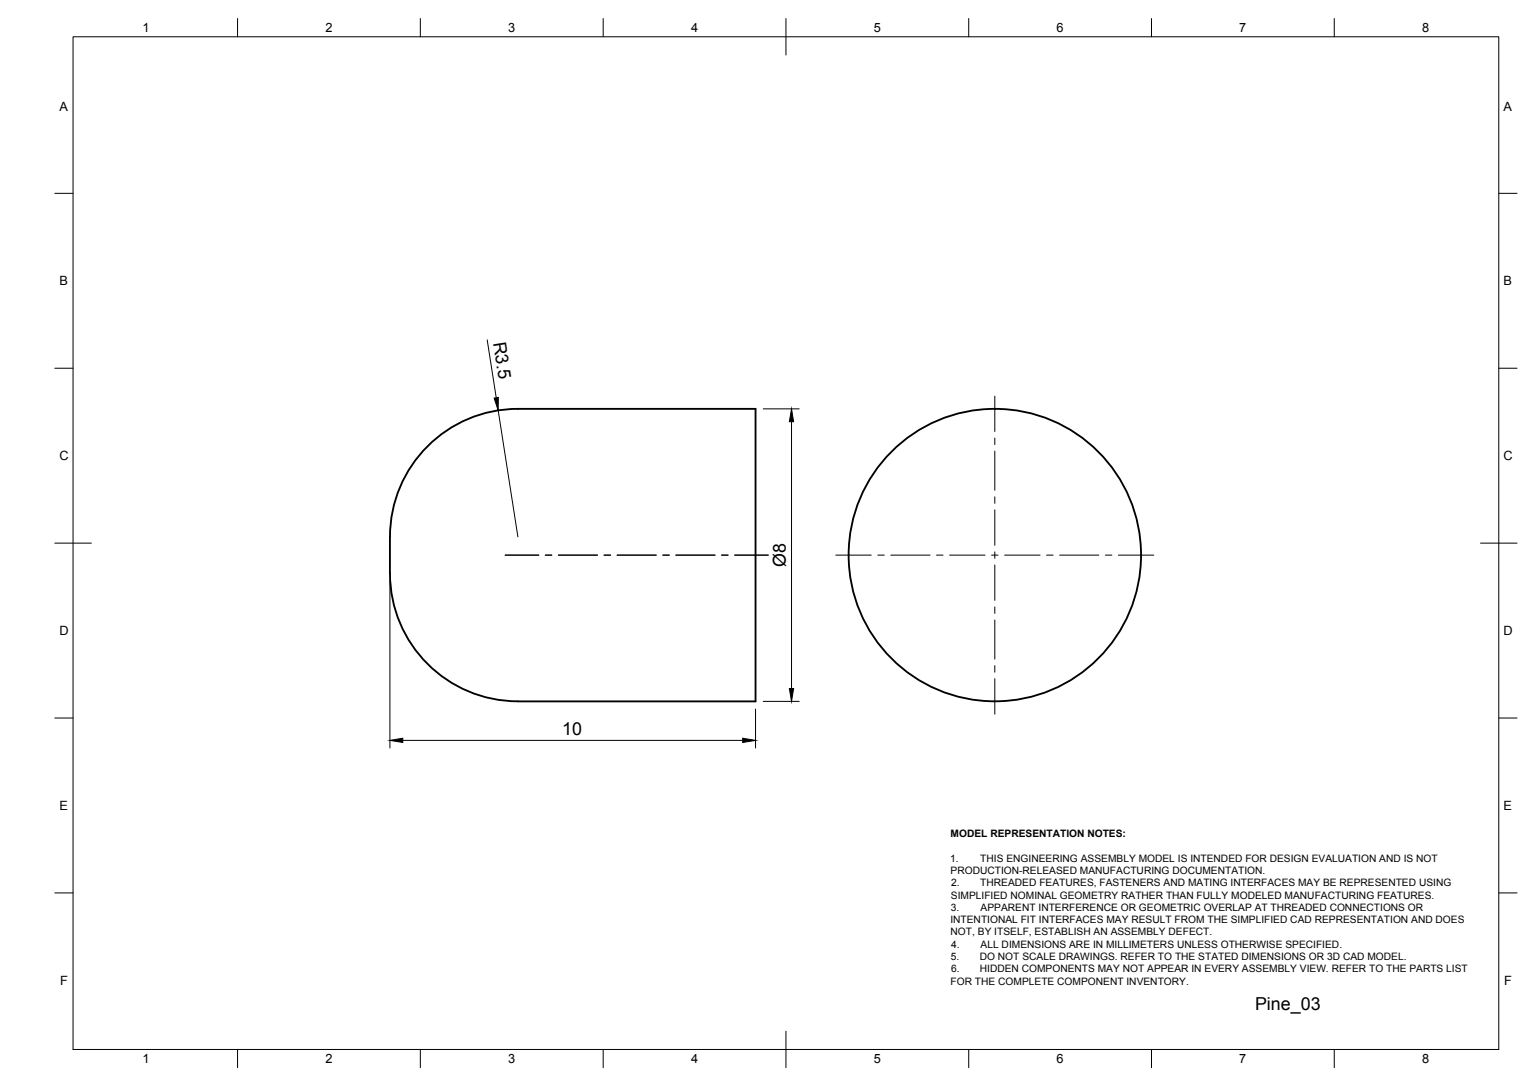
ISO-10303-21;
HEADER;
/* Generated by software containing ST-Developer
 * from STEP Tools, Inc. (www.steptools.com) 
 */

FILE_DESCRIPTION(
/* description */ (''),
/* implementation_level */ '2;1');

FILE_NAME(
/* name */ 'Pine_03.step',
/* time_stamp */ '2026-10-06T13:31:15-07:00',
/* author */ (''),
/* organization */ (''),
/* preprocessor_version */ 'ST-DEVELOPER v20.2',
/* originating_system */ 'Autodesk Translation Framework v15.15.0.0',
/* authorisation */ '');

FILE_SCHEMA (('AUTOMOTIVE_DESIGN { 1 0 10303 214 3 1 1 }'));
ENDSEC;

DATA;
#10=MECHANICAL_DESIGN_GEOMETRIC_PRESENTATION_REPRESENTATION('',(#84),#3154);
#49=(
BOUNDED_SURFACE()
B_SPLINE_SURFACE(2,2,((#2224,#2225,#2226,#2227,#2228,#2229,#2230,#2231,
#2232),(#2233,#2234,#2235,#2236,#2237,#2238,#2239,#2240,#2241),(#2242,#2243,
#2244,#2245,#2246,#2247,#2248,#2249,#2250)),.UNSPECIFIED.,.F.,.T.,.F.)
B_SPLINE_SURFACE_WITH_KNOTS((3,3),(3,2,2,2,3),(-6.11109985317371E-14,1.57079632679497),
(-3.14159265358979,-1.5707963267949,0.,1.5707963267949,3.14159265358979),
 .UNSPECIFIED.)
GEOMETRIC_REPRESENTATION_ITEM()
RATIONAL_B_SPLINE_SURFACE(((1.,0.707106781186548,1.,0.707106781186548,1.,
0.707106781186548,1.,0.707106781186548,1.),(0.707106781186505,0.49999999999997,
0.707106781186505,0.49999999999997,0.707106781186505,0.49999999999997,0.707106781186505,
0.49999999999997,0.707106781186505),(1.,0.707106781186548,1.,0.707106781186548,
1.,0.707106781186548,1.,0.707106781186548,1.)))
REPRESENTATION_ITEM('')
SURFACE()
);
#66=SHAPE_REPRESENTATION_RELATIONSHIP('SRR','None',#3194,#75);
#75=ADVANCED_BREP_SHAPE_REPRESENTATION('',(#93),#3150);
#84=STYLED_ITEM('',(#3243),#93);
#93=MANIFOLD_SOLID_BREP('Body1',#1086);
#114=PLANE('',#1246);
#115=PLANE('',#1247);
#157=CIRCLE('',#1240,3.99999999999999);
#158=CIRCLE('',#1241,3.49999999999999);
#159=CIRCLE('',#1242,0.49999999999999);
#160=CIRCLE('',#1243,3.99999999999999);
#161=CIRCLE('',#1245,3.99999999999999);
#202=FACE_OUTER_BOUND('',#266,.T.);
#203=FACE_OUTER_BOUND('',#267,.T.);
#204=FACE_OUTER_BOUND('',#268,.T.);
#205=FACE_OUTER_BOUND('',#269,.T.);
#266=EDGE_LOOP('',(#856,#857,#858,#859,#860));
#267=EDGE_LOOP('',(#861,#862,#863,#864,#865));
#268=EDGE_LOOP('',(#866));
#269=EDGE_LOOP('',(#867));
#332=LINE('',#2260,#398);
#398=VECTOR('',#1428,3.99999999999999);
#524=VERTEX_POINT('',#2251);
#525=VERTEX_POINT('',#2252);
#526=VERTEX_POINT('',#2254);
#527=VERTEX_POINT('',#2259);
#644=EDGE_CURVE('',#524,#525,#157,.T.);
#645=EDGE_CURVE('',#525,#526,#158,.T.);
#646=EDGE_CURVE('',#526,#526,#159,.T.);
#647=EDGE_CURVE('',#525,#524,#160,.T.);
#648=EDGE_CURVE('',#524,#527,#332,.T.);
#649=EDGE_CURVE('',#527,#527,#161,.T.);
#856=ORIENTED_EDGE('',*,*,#644,.T.);
#857=ORIENTED_EDGE('',*,*,#645,.T.);
#858=ORIENTED_EDGE('',*,*,#646,.T.);
#859=ORIENTED_EDGE('',*,*,#645,.F.);
#860=ORIENTED_EDGE('',*,*,#647,.T.);
#861=ORIENTED_EDGE('',*,*,#644,.F.);
#862=ORIENTED_EDGE('',*,*,#648,.T.);
#863=ORIENTED_EDGE('',*,*,#649,.T.);
#864=ORIENTED_EDGE('',*,*,#648,.F.);
#865=ORIENTED_EDGE('',*,*,#647,.F.);
#866=ORIENTED_EDGE('',*,*,#646,.F.);
#867=ORIENTED_EDGE('',*,*,#649,.F.);
#1016=CYLINDRICAL_SURFACE('',#1244,3.99999999999999);
#1053=ADVANCED_FACE('',(#202),#49,.F.);
#1054=ADVANCED_FACE('',(#203),#1016,.T.);
#1055=ADVANCED_FACE('',(#204),#114,.T.);
#1056=ADVANCED_FACE('',(#205),#115,.F.);
#1086=CLOSED_SHELL('',(#1053,#1054,#1055,#1056));
#1239=AXIS2_PLACEMENT_3D('',#2223,#1416,#1417);
#1240=AXIS2_PLACEMENT_3D('',#2253,#1418,#1419);
#1241=AXIS2_PLACEMENT_3D('',#2255,#1420,#1421);
#1242=AXIS2_PLACEMENT_3D('',#2256,#1422,#1423);
#1243=AXIS2_PLACEMENT_3D('',#2257,#1424,#1425);
#1244=AXIS2_PLACEMENT_3D('',#2258,#1426,#1427);
#1245=AXIS2_PLACEMENT_3D('',#2261,#1429,#1430);
#1246=AXIS2_PLACEMENT_3D('',#2262,#1431,#1432);
#1247=AXIS2_PLACEMENT_3D('',#2263,#1433,#1434);
#1416=DIRECTION('axis',(0.,0.,1.));
#1417=DIRECTION('refdir',(1.,0.,0.));
#1418=DIRECTION('center_axis',(1.,0.,0.));
#1419=DIRECTION('ref_axis',(0.,1.,0.));
#1420=DIRECTION('center_axis',(-5.11592739497909E-14,1.,1.22464679913998E-16));
#1421=DIRECTION('ref_axis',(-1.44328993201271E-14,-1.22464679914736E-16,
1.));
#1422=DIRECTION('center_axis',(-1.,0.,0.));
#1423=DIRECTION('ref_axis',(0.,1.,0.));
#1424=DIRECTION('center_axis',(1.,0.,0.));
#1425=DIRECTION('ref_axis',(0.,1.,0.));
#1426=DIRECTION('center_axis',(1.,0.,0.));
#1427=DIRECTION('ref_axis',(0.,1.,0.));
#1428=DIRECTION('',(-1.,0.,0.));
#1429=DIRECTION('center_axis',(1.,0.,0.));
#1430=DIRECTION('ref_axis',(0.,1.,0.));
#1431=DIRECTION('center_axis',(1.,0.,0.));
#1432=DIRECTION('ref_axis',(0.,1.,0.));
#1433=DIRECTION('center_axis',(1.,0.,0.));
#1434=DIRECTION('ref_axis',(0.,1.,0.));
#2223=CARTESIAN_POINT('',(0.,0.,0.));
#2224=CARTESIAN_POINT('Ctrl Pts',(23.4999999999997,2.05109366990699E-14,
324.));
#2225=CARTESIAN_POINT('Ctrl Pts',(23.4999999999999,-3.99999999999996,324.));
#2226=CARTESIAN_POINT('Ctrl Pts',(23.5,-3.99999999999997,320.));
#2227=CARTESIAN_POINT('Ctrl Pts',(23.5,-3.99999999999996,316.));
#2228=CARTESIAN_POINT('Ctrl Pts',(23.4999999999998,2.05109366990698E-14,
316.));
#2229=CARTESIAN_POINT('Ctrl Pts',(23.4999999999996,4.00000000000001,316.));
#2230=CARTESIAN_POINT('Ctrl Pts',(23.4999999999996,4.00000000000001,320.));
#2231=CARTESIAN_POINT('Ctrl Pts',(23.4999999999995,4.00000000000001,324.));
#2232=CARTESIAN_POINT('Ctrl Pts',(23.4999999999997,2.05109366990699E-14,
324.));
#2233=CARTESIAN_POINT('Ctrl Pts',(27.0000000000002,1.99568395523362E-13,
324.));
#2234=CARTESIAN_POINT('Ctrl Pts',(27.0000000000004,-4.00000000000003,324.));
#2235=CARTESIAN_POINT('Ctrl Pts',(27.0000000000004,-4.00000000000003,320.));
#2236=CARTESIAN_POINT('Ctrl Pts',(27.0000000000005,-4.00000000000003,316.));
#2237=CARTESIAN_POINT('Ctrl Pts',(27.0000000000003,1.99568395523362E-13,
316.));
#2238=CARTESIAN_POINT('Ctrl Pts',(27.0000000000001,4.00000000000043,316.));
#2239=CARTESIAN_POINT('Ctrl Pts',(27.,4.00000000000043,320.));
#2240=CARTESIAN_POINT('Ctrl Pts',(27.,4.00000000000043,324.));
#2241=CARTESIAN_POINT('Ctrl Pts',(27.0000000000002,1.99568395523362E-13,
324.));
#2242=CARTESIAN_POINT('Ctrl Pts',(27.,1.99568395523348E-13,320.5));
#2243=CARTESIAN_POINT('Ctrl Pts',(27.,-0.499999999999559,320.5));
#2244=CARTESIAN_POINT('Ctrl Pts',(27.,-0.499999999999559,320.));
#2245=CARTESIAN_POINT('Ctrl Pts',(27.,-0.499999999999559,319.5));
#2246=CARTESIAN_POINT('Ctrl Pts',(27.,1.99568395523348E-13,319.5));
#2247=CARTESIAN_POINT('Ctrl Pts',(27.,0.499999999999958,319.5));
#2248=CARTESIAN_POINT('Ctrl Pts',(27.,0.499999999999958,320.));
#2249=CARTESIAN_POINT('Ctrl Pts',(26.9999999999999,0.499999999999958,320.5));
#2250=CARTESIAN_POINT('Ctrl Pts',(27.,1.99568395523348E-13,320.5));
#2251=CARTESIAN_POINT('',(23.5,-3.99999999999999,320.));
#2252=CARTESIAN_POINT('',(23.5,2.00210779794253E-14,324.));
#2253=CARTESIAN_POINT('Origin',(23.5,0.,320.));
#2254=CARTESIAN_POINT('',(27.,-6.12323399573687E-17,320.5));
#2255=CARTESIAN_POINT('Origin',(23.5,2.04497043591234E-14,320.5));
#2256=CARTESIAN_POINT('Origin',(27.,0.,320.));
#2257=CARTESIAN_POINT('Origin',(23.5,0.,320.));
#2258=CARTESIAN_POINT('Origin',(2.,0.,320.));
#2259=CARTESIAN_POINT('',(17.,-3.99999999999999,320.));
#2260=CARTESIAN_POINT('',(2.,-3.99999999999999,320.));
#2261=CARTESIAN_POINT('Origin',(17.,0.,320.));
#2262=CARTESIAN_POINT('Origin',(27.,0.,320.));
#2263=CARTESIAN_POINT('Origin',(17.,0.,320.));
#3139=UNCERTAINTY_MEASURE_WITH_UNIT(LENGTH_MEASURE(0.01),#3155,
'DISTANCE_ACCURACY_VALUE',
'Maximum model space distance between geometric entities at asserted c
onnectivities');
#3143=UNCERTAINTY_MEASURE_WITH_UNIT(LENGTH_MEASURE(0.01),#3155,
'DISTANCE_ACCURACY_VALUE',
'Maximum model space distance between geometric entities at asserted c
onnectivities');
#3150=(
GEOMETRIC_REPRESENTATION_CONTEXT(3)
GLOBAL_UNCERTAINTY_ASSIGNED_CONTEXT((#3139))
GLOBAL_UNIT_ASSIGNED_CONTEXT((#3155,#3157,#3158))
REPRESENTATION_CONTEXT('','3D')
);
#3154=(
GEOMETRIC_REPRESENTATION_CONTEXT(3)
GLOBAL_UNCERTAINTY_ASSIGNED_CONTEXT((#3143))
GLOBAL_UNIT_ASSIGNED_CONTEXT((#3155,#3157,#3158))
REPRESENTATION_CONTEXT('','3D')
);
#3155=(
LENGTH_UNIT()
NAMED_UNIT(*)
SI_UNIT(.MILLI.,.METRE.)
);
#3157=(
NAMED_UNIT(*)
PLANE_ANGLE_UNIT()
SI_UNIT($,.RADIAN.)
);
#3158=(
NAMED_UNIT(*)
SI_UNIT($,.STERADIAN.)
SOLID_ANGLE_UNIT()
);
#3165=SHAPE_DEFINITION_REPRESENTATION(#3175,#3194);
#3175=PRODUCT_DEFINITION_SHAPE('',$,#3205);
#3194=SHAPE_REPRESENTATION('',(#1239),#3150);
#3198=PRODUCT_DEFINITION_CONTEXT('part definition',#3230,'design');
#3205=PRODUCT_DEFINITION('Pine_03','Pine_03',#3215,#3198);
#3215=PRODUCT_DEFINITION_FORMATION('',$,#3238);
#3230=APPLICATION_CONTEXT(
'Core Data for Automotive Mechanical Design Process');
#3231=PRODUCT_CONTEXT('part definition',#3230,'mechanical');
#3238=PRODUCT('Pine_03','Pine_03',$,(#3231));
#3243=PRESENTATION_STYLE_ASSIGNMENT((#3245));
#3245=SURFACE_STYLE_USAGE(.BOTH.,#3247);
#3247=SURFACE_SIDE_STYLE('',(#3249));
#3249=SURFACE_STYLE_FILL_AREA(#3251);
#3251=FILL_AREA_STYLE('Opaque(160,160,160)',(#3253));
#3253=FILL_AREA_STYLE_COLOUR('Opaque(160,160,160)',#3255);
#3255=COLOUR_RGB('Opaque(160,160,160)', 0.09019608, 0.27058824, 0.51372549);
ENDSEC;
END-ISO-10303-21;
